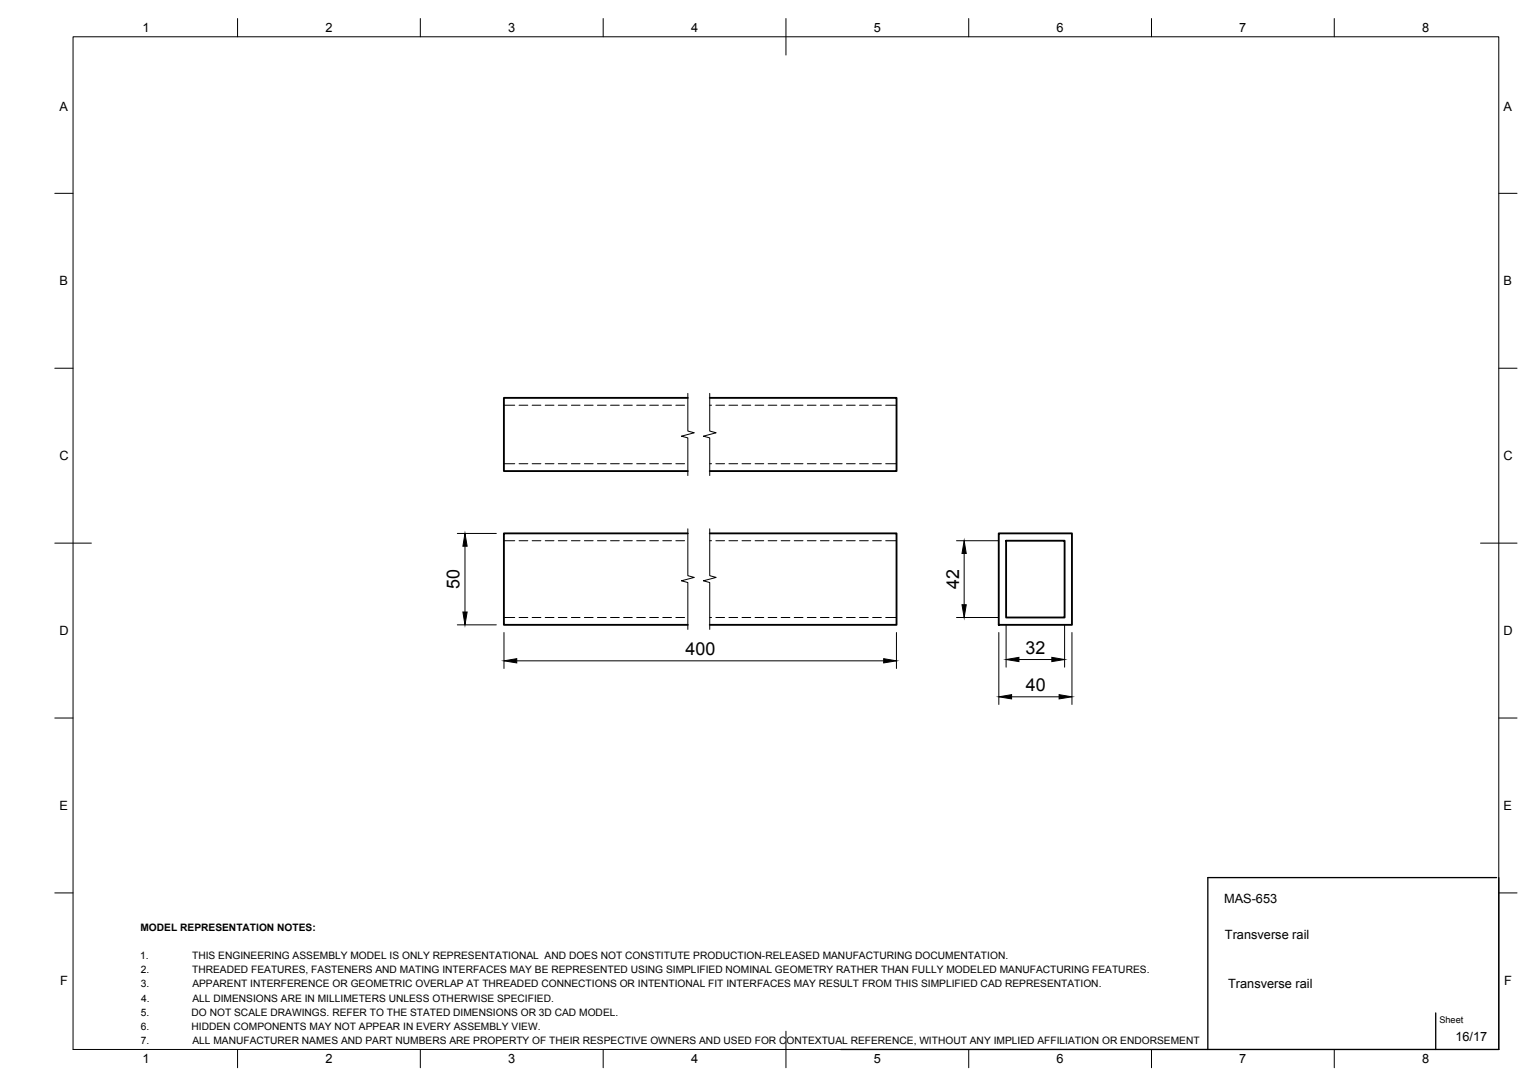
ISO-10303-21;
HEADER;
/* Generated by software containing ST-Developer
 * from STEP Tools, Inc. (www.steptools.com) 
 */

FILE_DESCRIPTION(
/* description */ ('Independent compact industrial fixture table, bolted aluminum worktop
 on connected adjustable support base. Whole-mm nominal dimensions. No
 load rating assigned.'),
/* implementation_level */ '2;1');

FILE_NAME(
/* name */ 'Transverse rail.step',
/* time_stamp */ '2026-11-07T17:47:58-08:00',
/* author */ (''),
/* organization */ (''),
/* preprocessor_version */ 'ST-DEVELOPER v20.2',
/* originating_system */ 'Autodesk Translation Framework v15.17.0.0',
/* authorisation */ '');

FILE_SCHEMA (('AUTOMOTIVE_DESIGN { 1 0 10303 214 3 1 1 }'));
ENDSEC;

DATA;
#10=MECHANICAL_DESIGN_GEOMETRIC_PRESENTATION_REPRESENTATION('',(#2251),#97475);
#2213=SHAPE_REPRESENTATION_RELATIONSHIP('SRR','None',#97606,#2232);
#2232=ADVANCED_BREP_SHAPE_REPRESENTATION('',(#2270),#97456);
#2251=STYLED_ITEM('',(#97718),#2270);
#2270=MANIFOLD_SOLID_BREP('Body1',#21812);
#2302=FACE_BOUND('',#3730,.T.);
#2303=FACE_BOUND('',#3732,.T.);
#2389=PLANE('',#22072);
#2390=PLANE('',#22073);
#2391=PLANE('',#22074);
#2392=PLANE('',#22075);
#2393=PLANE('',#22076);
#2394=PLANE('',#22077);
#2395=PLANE('',#22078);
#2396=PLANE('',#22079);
#2397=PLANE('',#22080);
#2398=PLANE('',#22081);
#2553=FACE_OUTER_BOUND('',#3721,.T.);
#2554=FACE_OUTER_BOUND('',#3722,.T.);
#2555=FACE_OUTER_BOUND('',#3723,.T.);
#2556=FACE_OUTER_BOUND('',#3724,.T.);
#2557=FACE_OUTER_BOUND('',#3725,.T.);
#2558=FACE_OUTER_BOUND('',#3726,.T.);
#2559=FACE_OUTER_BOUND('',#3727,.T.);
#2560=FACE_OUTER_BOUND('',#3728,.T.);
#2561=FACE_OUTER_BOUND('',#3729,.T.);
#2562=FACE_OUTER_BOUND('',#3731,.T.);
#3721=EDGE_LOOP('',(#13196,#13197,#13198,#13199));
#3722=EDGE_LOOP('',(#13200,#13201,#13202,#13203));
#3723=EDGE_LOOP('',(#13204,#13205,#13206,#13207));
#3724=EDGE_LOOP('',(#13208,#13209,#13210,#13211));
#3725=EDGE_LOOP('',(#13212,#13213,#13214,#13215));
#3726=EDGE_LOOP('',(#13216,#13217,#13218,#13219));
#3727=EDGE_LOOP('',(#13220,#13221,#13222,#13223));
#3728=EDGE_LOOP('',(#13224,#13225,#13226,#13227));
#3729=EDGE_LOOP('',(#13228,#13229,#13230,#13231));
#3730=EDGE_LOOP('',(#13232,#13233,#13234,#13235));
#3731=EDGE_LOOP('',(#13236,#13237,#13238,#13239));
#3732=EDGE_LOOP('',(#13240,#13241,#13242,#13243));
#4966=LINE('',#27733,#6180);
#4967=LINE('',#27735,#6181);
#4968=LINE('',#27737,#6182);
#4969=LINE('',#27738,#6183);
#4970=LINE('',#27741,#6184);
#4971=LINE('',#27743,#6185);
#4972=LINE('',#27744,#6186);
#4973=LINE('',#27747,#6187);
#4974=LINE('',#27749,#6188);
#4975=LINE('',#27750,#6189);
#4976=LINE('',#27752,#6190);
#4977=LINE('',#27753,#6191);
#4978=LINE('',#27757,#6192);
#4979=LINE('',#27759,#6193);
#4980=LINE('',#27761,#6194);
#4981=LINE('',#27762,#6195);
#4982=LINE('',#27765,#6196);
#4983=LINE('',#27767,#6197);
#4984=LINE('',#27768,#6198);
#4985=LINE('',#27771,#6199);
#4986=LINE('',#27773,#6200);
#4987=LINE('',#27774,#6201);
#4988=LINE('',#27776,#6202);
#4989=LINE('',#27777,#6203);
#6180=VECTOR('',#23598,10.);
#6181=VECTOR('',#23599,10.);
#6182=VECTOR('',#23600,10.);
#6183=VECTOR('',#23601,10.);
#6184=VECTOR('',#23604,10.);
#6185=VECTOR('',#23605,10.);
#6186=VECTOR('',#23606,10.);
#6187=VECTOR('',#23609,10.);
#6188=VECTOR('',#23610,10.);
#6189=VECTOR('',#23611,10.);
#6190=VECTOR('',#23614,10.);
#6191=VECTOR('',#23615,10.);
#6192=VECTOR('',#23618,10.);
#6193=VECTOR('',#23619,10.);
#6194=VECTOR('',#23620,10.);
#6195=VECTOR('',#23621,10.);
#6196=VECTOR('',#23624,10.);
#6197=VECTOR('',#23625,10.);
#6198=VECTOR('',#23626,10.);
#6199=VECTOR('',#23629,10.);
#6200=VECTOR('',#23630,10.);
#6201=VECTOR('',#23631,10.);
#6202=VECTOR('',#23634,10.);
#6203=VECTOR('',#23635,10.);
#7641=VERTEX_POINT('',#27731);
#7642=VERTEX_POINT('',#27732);
#7643=VERTEX_POINT('',#27734);
#7644=VERTEX_POINT('',#27736);
#7645=VERTEX_POINT('',#27740);
#7646=VERTEX_POINT('',#27742);
#7647=VERTEX_POINT('',#27746);
#7648=VERTEX_POINT('',#27748);
#7649=VERTEX_POINT('',#27755);
#7650=VERTEX_POINT('',#27756);
#7651=VERTEX_POINT('',#27758);
#7652=VERTEX_POINT('',#27760);
#7653=VERTEX_POINT('',#27764);
#7654=VERTEX_POINT('',#27766);
#7655=VERTEX_POINT('',#27770);
#7656=VERTEX_POINT('',#27772);
#9855=EDGE_CURVE('',#7641,#7642,#4966,.T.);
#9856=EDGE_CURVE('',#7642,#7643,#4967,.T.);
#9857=EDGE_CURVE('',#7644,#7643,#4968,.T.);
#9858=EDGE_CURVE('',#7641,#7644,#4969,.T.);
#9859=EDGE_CURVE('',#7645,#7641,#4970,.T.);
#9860=EDGE_CURVE('',#7646,#7644,#4971,.T.);
#9861=EDGE_CURVE('',#7645,#7646,#4972,.T.);
#9862=EDGE_CURVE('',#7647,#7645,#4973,.T.);
#9863=EDGE_CURVE('',#7648,#7646,#4974,.T.);
#9864=EDGE_CURVE('',#7647,#7648,#4975,.T.);
#9865=EDGE_CURVE('',#7642,#7647,#4976,.T.);
#9866=EDGE_CURVE('',#7643,#7648,#4977,.T.);
#9867=EDGE_CURVE('',#7649,#7650,#4978,.T.);
#9868=EDGE_CURVE('',#7650,#7651,#4979,.T.);
#9869=EDGE_CURVE('',#7652,#7651,#4980,.T.);
#9870=EDGE_CURVE('',#7649,#7652,#4981,.T.);
#9871=EDGE_CURVE('',#7653,#7649,#4982,.T.);
#9872=EDGE_CURVE('',#7654,#7652,#4983,.T.);
#9873=EDGE_CURVE('',#7653,#7654,#4984,.T.);
#9874=EDGE_CURVE('',#7655,#7653,#4985,.T.);
#9875=EDGE_CURVE('',#7656,#7654,#4986,.T.);
#9876=EDGE_CURVE('',#7655,#7656,#4987,.T.);
#9877=EDGE_CURVE('',#7650,#7655,#4988,.T.);
#9878=EDGE_CURVE('',#7651,#7656,#4989,.T.);
#13196=ORIENTED_EDGE('',*,*,#9855,.T.);
#13197=ORIENTED_EDGE('',*,*,#9856,.T.);
#13198=ORIENTED_EDGE('',*,*,#9857,.F.);
#13199=ORIENTED_EDGE('',*,*,#9858,.F.);
#13200=ORIENTED_EDGE('',*,*,#9859,.T.);
#13201=ORIENTED_EDGE('',*,*,#9858,.T.);
#13202=ORIENTED_EDGE('',*,*,#9860,.F.);
#13203=ORIENTED_EDGE('',*,*,#9861,.F.);
#13204=ORIENTED_EDGE('',*,*,#9862,.T.);
#13205=ORIENTED_EDGE('',*,*,#9861,.T.);
#13206=ORIENTED_EDGE('',*,*,#9863,.F.);
#13207=ORIENTED_EDGE('',*,*,#9864,.F.);
#13208=ORIENTED_EDGE('',*,*,#9865,.T.);
#13209=ORIENTED_EDGE('',*,*,#9864,.T.);
#13210=ORIENTED_EDGE('',*,*,#9866,.F.);
#13211=ORIENTED_EDGE('',*,*,#9856,.F.);
#13212=ORIENTED_EDGE('',*,*,#9867,.T.);
#13213=ORIENTED_EDGE('',*,*,#9868,.T.);
#13214=ORIENTED_EDGE('',*,*,#9869,.F.);
#13215=ORIENTED_EDGE('',*,*,#9870,.F.);
#13216=ORIENTED_EDGE('',*,*,#9871,.T.);
#13217=ORIENTED_EDGE('',*,*,#9870,.T.);
#13218=ORIENTED_EDGE('',*,*,#9872,.F.);
#13219=ORIENTED_EDGE('',*,*,#9873,.F.);
#13220=ORIENTED_EDGE('',*,*,#9874,.T.);
#13221=ORIENTED_EDGE('',*,*,#9873,.T.);
#13222=ORIENTED_EDGE('',*,*,#9875,.F.);
#13223=ORIENTED_EDGE('',*,*,#9876,.F.);
#13224=ORIENTED_EDGE('',*,*,#9877,.T.);
#13225=ORIENTED_EDGE('',*,*,#9876,.T.);
#13226=ORIENTED_EDGE('',*,*,#9878,.F.);
#13227=ORIENTED_EDGE('',*,*,#9868,.F.);
#13228=ORIENTED_EDGE('',*,*,#9878,.T.);
#13229=ORIENTED_EDGE('',*,*,#9875,.T.);
#13230=ORIENTED_EDGE('',*,*,#9872,.T.);
#13231=ORIENTED_EDGE('',*,*,#9869,.T.);
#13232=ORIENTED_EDGE('',*,*,#9866,.T.);
#13233=ORIENTED_EDGE('',*,*,#9863,.T.);
#13234=ORIENTED_EDGE('',*,*,#9860,.T.);
#13235=ORIENTED_EDGE('',*,*,#9857,.T.);
#13236=ORIENTED_EDGE('',*,*,#9877,.F.);
#13237=ORIENTED_EDGE('',*,*,#9867,.F.);
#13238=ORIENTED_EDGE('',*,*,#9871,.F.);
#13239=ORIENTED_EDGE('',*,*,#9874,.F.);
#13240=ORIENTED_EDGE('',*,*,#9865,.F.);
#13241=ORIENTED_EDGE('',*,*,#9855,.F.);
#13242=ORIENTED_EDGE('',*,*,#9859,.F.);
#13243=ORIENTED_EDGE('',*,*,#9862,.F.);
#20673=ADVANCED_FACE('',(#2553),#2389,.T.);
#20674=ADVANCED_FACE('',(#2554),#2390,.T.);
#20675=ADVANCED_FACE('',(#2555),#2391,.T.);
#20676=ADVANCED_FACE('',(#2556),#2392,.T.);
#20677=ADVANCED_FACE('',(#2557),#2393,.T.);
#20678=ADVANCED_FACE('',(#2558),#2394,.T.);
#20679=ADVANCED_FACE('',(#2559),#2395,.T.);
#20680=ADVANCED_FACE('',(#2560),#2396,.T.);
#20681=ADVANCED_FACE('',(#2561,#2302),#2397,.T.);
#20682=ADVANCED_FACE('',(#2562,#2303),#2398,.F.);
#21812=CLOSED_SHELL('',(#20673,#20674,#20675,#20676,#20677,#20678,#20679,
#20680,#20681,#20682));
#22071=AXIS2_PLACEMENT_3D('',#27729,#23594,#23595);
#22072=AXIS2_PLACEMENT_3D('',#27730,#23596,#23597);
#22073=AXIS2_PLACEMENT_3D('',#27739,#23602,#23603);
#22074=AXIS2_PLACEMENT_3D('',#27745,#23607,#23608);
#22075=AXIS2_PLACEMENT_3D('',#27751,#23612,#23613);
#22076=AXIS2_PLACEMENT_3D('',#27754,#23616,#23617);
#22077=AXIS2_PLACEMENT_3D('',#27763,#23622,#23623);
#22078=AXIS2_PLACEMENT_3D('',#27769,#23627,#23628);
#22079=AXIS2_PLACEMENT_3D('',#27775,#23632,#23633);
#22080=AXIS2_PLACEMENT_3D('',#27778,#23636,#23637);
#22081=AXIS2_PLACEMENT_3D('',#27779,#23638,#23639);
#23594=DIRECTION('axis',(0.,0.,1.));
#23595=DIRECTION('refdir',(1.,0.,0.));
#23596=DIRECTION('center_axis',(0.,1.,0.));
#23597=DIRECTION('ref_axis',(-1.,0.,0.));
#23598=DIRECTION('',(-1.,0.,0.));
#23599=DIRECTION('',(0.,0.,1.));
#23600=DIRECTION('',(-1.,0.,0.));
#23601=DIRECTION('',(0.,0.,1.));
#23602=DIRECTION('center_axis',(-1.,0.,0.));
#23603=DIRECTION('ref_axis',(0.,-1.,0.));
#23604=DIRECTION('',(0.,-1.,0.));
#23605=DIRECTION('',(0.,-1.,0.));
#23606=DIRECTION('',(0.,0.,1.));
#23607=DIRECTION('center_axis',(0.,-1.,0.));
#23608=DIRECTION('ref_axis',(1.,0.,0.));
#23609=DIRECTION('',(1.,0.,0.));
#23610=DIRECTION('',(1.,0.,0.));
#23611=DIRECTION('',(0.,0.,1.));
#23612=DIRECTION('center_axis',(1.,0.,0.));
#23613=DIRECTION('ref_axis',(0.,1.,0.));
#23614=DIRECTION('',(0.,1.,0.));
#23615=DIRECTION('',(0.,1.,0.));
#23616=DIRECTION('center_axis',(0.,1.,0.));
#23617=DIRECTION('ref_axis',(-1.,0.,0.));
#23618=DIRECTION('',(-1.,0.,0.));
#23619=DIRECTION('',(0.,0.,1.));
#23620=DIRECTION('',(-1.,0.,0.));
#23621=DIRECTION('',(0.,0.,1.));
#23622=DIRECTION('center_axis',(1.,0.,0.));
#23623=DIRECTION('ref_axis',(0.,1.,0.));
#23624=DIRECTION('',(0.,1.,0.));
#23625=DIRECTION('',(0.,1.,0.));
#23626=DIRECTION('',(0.,0.,1.));
#23627=DIRECTION('center_axis',(0.,-1.,0.));
#23628=DIRECTION('ref_axis',(1.,0.,0.));
#23629=DIRECTION('',(1.,0.,0.));
#23630=DIRECTION('',(1.,0.,0.));
#23631=DIRECTION('',(0.,0.,1.));
#23632=DIRECTION('center_axis',(-1.,0.,0.));
#23633=DIRECTION('ref_axis',(0.,-1.,0.));
#23634=DIRECTION('',(0.,-1.,0.));
#23635=DIRECTION('',(0.,-1.,0.));
#23636=DIRECTION('center_axis',(0.,0.,1.));
#23637=DIRECTION('ref_axis',(1.,0.,0.));
#23638=DIRECTION('center_axis',(0.,0.,1.));
#23639=DIRECTION('ref_axis',(1.,0.,0.));
#27729=CARTESIAN_POINT('',(0.,0.,0.));
#27730=CARTESIAN_POINT('Origin',(16.,-21.,0.));
#27731=CARTESIAN_POINT('',(16.,-21.,0.));
#27732=CARTESIAN_POINT('',(-16.,-21.,0.));
#27733=CARTESIAN_POINT('',(-16.,-21.,0.));
#27734=CARTESIAN_POINT('',(-16.,-21.,400.));
#27735=CARTESIAN_POINT('',(-16.,-21.,0.));
#27736=CARTESIAN_POINT('',(16.,-21.,400.));
#27737=CARTESIAN_POINT('',(-16.,-21.,400.));
#27738=CARTESIAN_POINT('',(16.,-21.,0.));
#27739=CARTESIAN_POINT('Origin',(16.,21.,0.));
#27740=CARTESIAN_POINT('',(16.,21.,0.));
#27741=CARTESIAN_POINT('',(16.,-21.,0.));
#27742=CARTESIAN_POINT('',(16.,21.,400.));
#27743=CARTESIAN_POINT('',(16.,-21.,400.));
#27744=CARTESIAN_POINT('',(16.,21.,0.));
#27745=CARTESIAN_POINT('Origin',(-16.,21.,0.));
#27746=CARTESIAN_POINT('',(-16.,21.,0.));
#27747=CARTESIAN_POINT('',(16.,21.,0.));
#27748=CARTESIAN_POINT('',(-16.,21.,400.));
#27749=CARTESIAN_POINT('',(16.,21.,400.));
#27750=CARTESIAN_POINT('',(-16.,21.,0.));
#27751=CARTESIAN_POINT('Origin',(-16.,-21.,0.));
#27752=CARTESIAN_POINT('',(-16.,21.,0.));
#27753=CARTESIAN_POINT('',(-16.,21.,400.));
#27754=CARTESIAN_POINT('Origin',(20.,25.,0.));
#27755=CARTESIAN_POINT('',(20.,25.,0.));
#27756=CARTESIAN_POINT('',(-20.,25.,0.));
#27757=CARTESIAN_POINT('',(20.,25.,0.));
#27758=CARTESIAN_POINT('',(-20.,25.,400.));
#27759=CARTESIAN_POINT('',(-20.,25.,0.));
#27760=CARTESIAN_POINT('',(20.,25.,400.));
#27761=CARTESIAN_POINT('',(20.,25.,400.));
#27762=CARTESIAN_POINT('',(20.,25.,0.));
#27763=CARTESIAN_POINT('Origin',(20.,-25.,0.));
#27764=CARTESIAN_POINT('',(20.,-25.,0.));
#27765=CARTESIAN_POINT('',(20.,-25.,0.));
#27766=CARTESIAN_POINT('',(20.,-25.,400.));
#27767=CARTESIAN_POINT('',(20.,-25.,400.));
#27768=CARTESIAN_POINT('',(20.,-25.,0.));
#27769=CARTESIAN_POINT('Origin',(-20.,-25.,0.));
#27770=CARTESIAN_POINT('',(-20.,-25.,0.));
#27771=CARTESIAN_POINT('',(-20.,-25.,0.));
#27772=CARTESIAN_POINT('',(-20.,-25.,400.));
#27773=CARTESIAN_POINT('',(-20.,-25.,400.));
#27774=CARTESIAN_POINT('',(-20.,-25.,0.));
#27775=CARTESIAN_POINT('Origin',(-20.,25.,0.));
#27776=CARTESIAN_POINT('',(-20.,25.,0.));
#27777=CARTESIAN_POINT('',(-20.,25.,400.));
#27778=CARTESIAN_POINT('Origin',(0.,0.,400.));
#27779=CARTESIAN_POINT('Origin',(0.,0.,0.));
#97433=UNCERTAINTY_MEASURE_WITH_UNIT(LENGTH_MEASURE(0.01),#97476,
'DISTANCE_ACCURACY_VALUE',
'Maximum model space distance between geometric entities at asserted c
onnectivities');
#97452=UNCERTAINTY_MEASURE_WITH_UNIT(LENGTH_MEASURE(0.01),#97476,
'DISTANCE_ACCURACY_VALUE',
'Maximum model space distance between geometric entities at asserted c
onnectivities');
#97456=(
GEOMETRIC_REPRESENTATION_CONTEXT(3)
GLOBAL_UNCERTAINTY_ASSIGNED_CONTEXT((#97433))
GLOBAL_UNIT_ASSIGNED_CONTEXT((#97476,#97478,#97479))
REPRESENTATION_CONTEXT('','3D')
);
#97475=(
GEOMETRIC_REPRESENTATION_CONTEXT(3)
GLOBAL_UNCERTAINTY_ASSIGNED_CONTEXT((#97452))
GLOBAL_UNIT_ASSIGNED_CONTEXT((#97476,#97478,#97479))
REPRESENTATION_CONTEXT('','3D')
);
#97476=(
LENGTH_UNIT()
NAMED_UNIT(*)
SI_UNIT(.MILLI.,.METRE.)
);
#97478=(
NAMED_UNIT(*)
PLANE_ANGLE_UNIT()
SI_UNIT($,.RADIAN.)
);
#97479=(
NAMED_UNIT(*)
SI_UNIT($,.STERADIAN.)
SOLID_ANGLE_UNIT()
);
#97483=SHAPE_DEFINITION_REPRESENTATION(#97505,#97606);
#97505=PRODUCT_DEFINITION_SHAPE('',$,#97629);
#97606=SHAPE_REPRESENTATION('',(#22071),#97456);
#97625=PRODUCT_DEFINITION_CONTEXT('part definition',#97693,'design');
#97629=PRODUCT_DEFINITION('Transverse rail','Transverse rail',#97651,#97625);
#97651=PRODUCT_DEFINITION_FORMATION('',$,#97698);
#97693=APPLICATION_CONTEXT(
'Core Data for Automotive Mechanical Design Process');
#97694=PRODUCT_CONTEXT('part definition',#97693,'mechanical');
#97698=PRODUCT('Transverse rail','Transverse rail',
'Steel rectangular hollow section, 50 x 40 mm, 4 mm wall. Square cut e
nds; weld to adjoining rails and corner plates.',(#97694));
#97718=PRESENTATION_STYLE_ASSIGNMENT((#97725));
#97725=SURFACE_STYLE_USAGE(.BOTH.,#97732);
#97732=SURFACE_SIDE_STYLE('',(#97739));
#97739=SURFACE_STYLE_FILL_AREA(#97746);
#97746=FILL_AREA_STYLE('Dark blue',(#97753));
#97753=FILL_AREA_STYLE_COLOUR('Dark blue',#97760);
#97760=COLOUR_RGB('Dark blue',0.0901960784313725,0.270588235294118,0.513725490196078);
ENDSEC;
END-ISO-10303-21;
